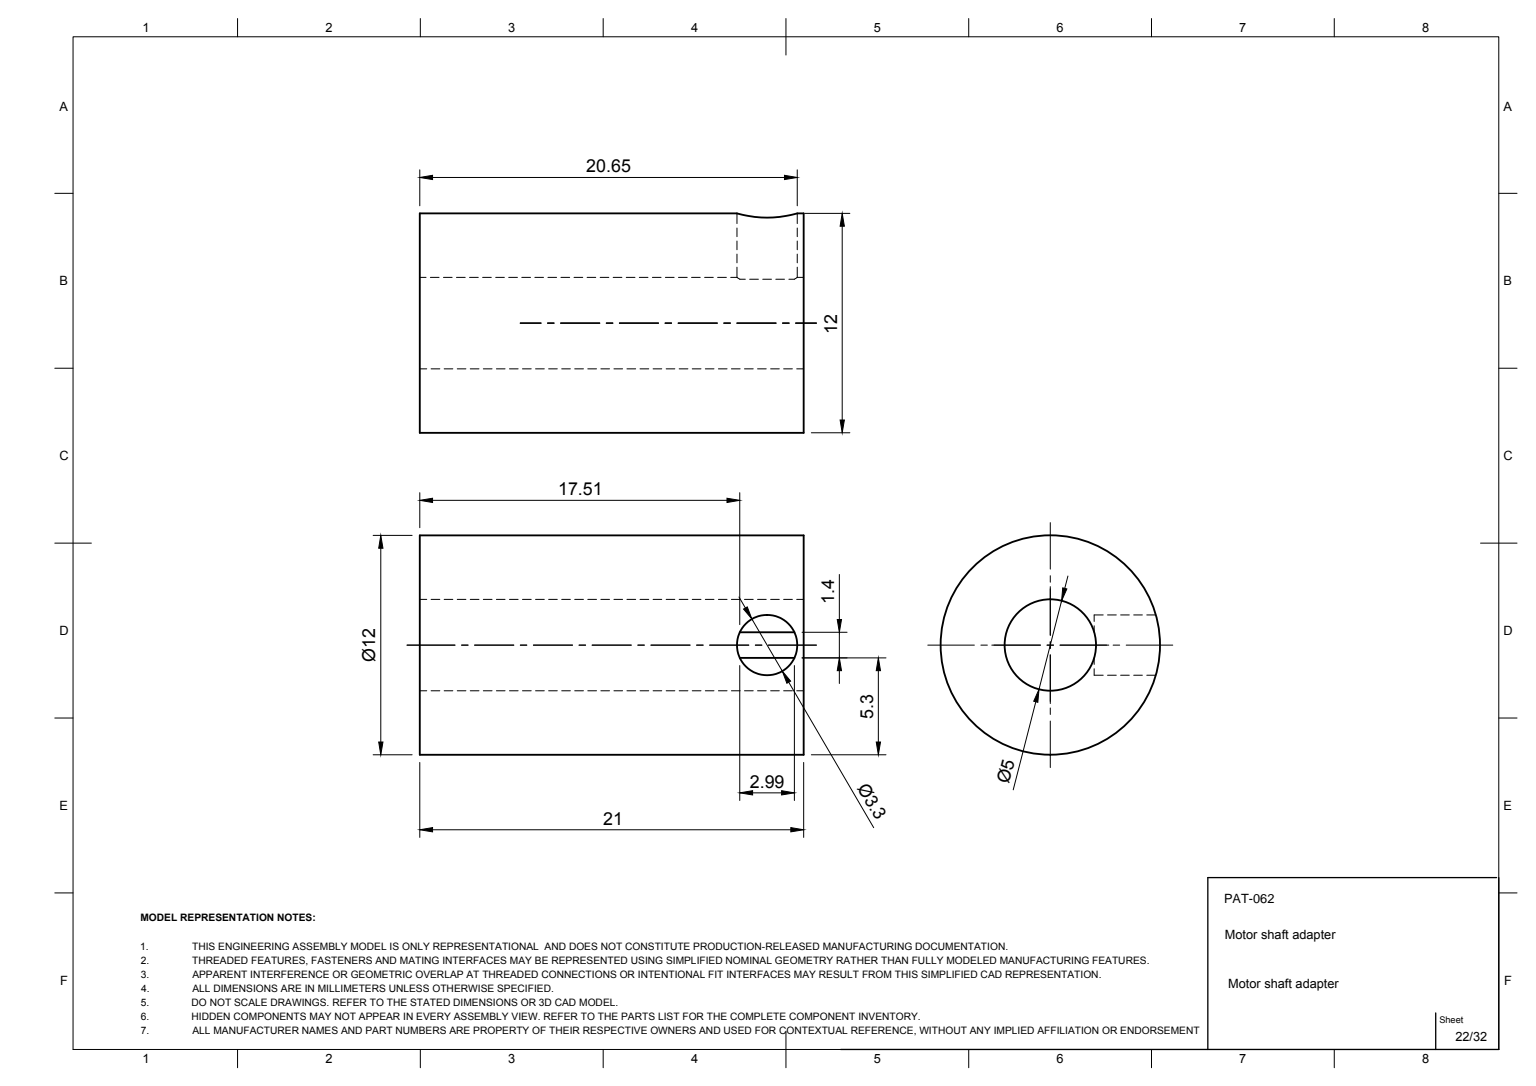
ISO-10303-21;
HEADER;
/* Generated by software containing ST-Developer
 * from STEP Tools, Inc. (www.steptools.com) 
 */

FILE_DESCRIPTION(
/* description */ ('Jaw-coupled motor to shaft test stand'),
/* implementation_level */ '2;1');

FILE_NAME(
/* name */ 'Motor shaft adapter.step',
/* time_stamp */ '2026-10-27T10:46:06-07:00',
/* author */ (''),
/* organization */ (''),
/* preprocessor_version */ 'ST-DEVELOPER v20.2',
/* originating_system */ 'Autodesk Translation Framework v15.17.0.0',
/* authorisation */ '');

FILE_SCHEMA (('AUTOMOTIVE_DESIGN { 1 0 10303 214 3 1 1 }'));
ENDSEC;

DATA;
#10=MECHANICAL_DESIGN_GEOMETRIC_PRESENTATION_REPRESENTATION('',(#361),#19361);
#251=B_SPLINE_CURVE_WITH_KNOTS('',3,(#16870,#16871,#16872,#16873,#16874,
#16875,#16876,#16877,#16878,#16879),.UNSPECIFIED.,.F.,.F.,(4,2,2,2,4),(0.705412572778712,
0.711709336094043,0.776040013313971,0.840370690533898,0.846667453849229),
 .UNSPECIFIED.);
#252=B_SPLINE_CURVE_WITH_KNOTS('',3,(#16885,#16886,#16887,#16888,#16889,
#16890,#16891,#16892,#16893,#16894,#16895,#16896,#16897,#16898,#16899,#16900,
#16901,#16902),.UNSPECIFIED.,.F.,.F.,(4,2,2,2,2,2,2,2,4),(0.,0.0625085224334669,
0.125017044866934,0.187512605393579,0.250008165920225,0.312503726446871,
0.374999286973516,0.437507809406983,0.50001633184045),.UNSPECIFIED.);
#253=B_SPLINE_CURVE_WITH_KNOTS('',3,(#16903,#16904,#16905,#16906,#16907,
#16908,#16909,#16910,#16911,#16912,#16913,#16914,#16915,#16916,#16917,#16918,
#16919,#16920),.UNSPECIFIED.,.F.,.F.,(4,2,2,2,2,2,2,2,4),(0.50001633184045,
0.562524854273917,0.625033376707384,0.687528937234029,0.750024497760675,
0.81252005828732,0.875015618813966,0.937524141247433,1.0000326636809),
 .UNSPECIFIED.);
#254=B_SPLINE_CURVE_WITH_KNOTS('',3,(#16923,#16924,#16925,#16926,#16927,
#16928,#16929,#16930,#16931,#16932),.UNSPECIFIED.,.F.,.F.,(4,2,2,2,4),(0.188052563902732,
0.194349327218063,0.25868000443799,0.323010681657918,0.329307444973249),
 .UNSPECIFIED.);
#296=SHAPE_REPRESENTATION_RELATIONSHIP('SRR','None',#19512,#328);
#328=ADVANCED_BREP_SHAPE_REPRESENTATION('',(#392),#19348);
#361=STYLED_ITEM('',(#19746),#392);
#392=MANIFOLD_SOLID_BREP('Body1',#11007);
#485=FACE_BOUND('',#1942,.T.);
#486=FACE_BOUND('',#1944,.T.);
#487=FACE_BOUND('',#1946,.T.);
#488=FACE_BOUND('',#1948,.T.);
#662=PLANE('',#11767);
#663=PLANE('',#11772);
#664=PLANE('',#11779);
#665=PLANE('',#11780);
#1236=FACE_OUTER_BOUND('',#1938,.T.);
#1237=FACE_OUTER_BOUND('',#1939,.T.);
#1238=FACE_OUTER_BOUND('',#1940,.T.);
#1239=FACE_OUTER_BOUND('',#1941,.T.);
#1240=FACE_OUTER_BOUND('',#1943,.T.);
#1241=FACE_OUTER_BOUND('',#1945,.T.);
#1242=FACE_OUTER_BOUND('',#1947,.T.);
#1938=EDGE_LOOP('',(#8254,#8255));
#1939=EDGE_LOOP('',(#8256,#8257,#8258,#8259,#8260,#8261,#8262,#8263,#8264));
#1940=EDGE_LOOP('',(#8265,#8266,#8267));
#1941=EDGE_LOOP('',(#8268,#8269,#8270,#8271));
#1942=EDGE_LOOP('',(#8272,#8273,#8274,#8275));
#1943=EDGE_LOOP('',(#8276,#8277,#8278,#8279));
#1944=EDGE_LOOP('',(#8280,#8281));
#1945=EDGE_LOOP('',(#8282));
#1946=EDGE_LOOP('',(#8283));
#1947=EDGE_LOOP('',(#8284));
#1948=EDGE_LOOP('',(#8285));
#2677=LINE('',#16866,#3830);
#2678=LINE('',#16883,#3831);
#2679=LINE('',#16934,#3832);
#2680=LINE('',#16939,#3833);
#2681=LINE('',#16945,#3834);
#3830=VECTOR('',#13432,1.);
#3831=VECTOR('',#13439,0.165);
#3832=VECTOR('',#13444,1.);
#3833=VECTOR('',#13449,0.25);
#3834=VECTOR('',#13456,0.6);
#4809=CIRCLE('',#11768,0.165);
#4810=CIRCLE('',#11770,0.165);
#4811=CIRCLE('',#11771,0.165);
#4812=CIRCLE('',#11774,0.25);
#4813=CIRCLE('',#11775,0.25);
#4814=CIRCLE('',#11777,0.6);
#4815=CIRCLE('',#11778,0.6);
#5251=VERTEX_POINT('',#16864);
#5252=VERTEX_POINT('',#16865);
#5253=VERTEX_POINT('',#16869);
#5254=VERTEX_POINT('',#16880);
#5255=VERTEX_POINT('',#16882);
#5256=VERTEX_POINT('',#16884);
#5257=VERTEX_POINT('',#16921);
#5258=VERTEX_POINT('',#16936);
#5259=VERTEX_POINT('',#16938);
#5260=VERTEX_POINT('',#16942);
#5261=VERTEX_POINT('',#16944);
#6338=EDGE_CURVE('',#5251,#5252,#2677,.T.);
#6339=EDGE_CURVE('',#5251,#5252,#4809,.T.);
#6340=EDGE_CURVE('',#5253,#5251,#251,.T.);
#6341=EDGE_CURVE('',#5254,#5253,#4810,.T.);
#6342=EDGE_CURVE('',#5254,#5255,#2678,.T.);
#6343=EDGE_CURVE('',#5256,#5255,#252,.T.);
#6344=EDGE_CURVE('',#5255,#5256,#253,.T.);
#6345=EDGE_CURVE('',#5257,#5254,#4811,.T.);
#6346=EDGE_CURVE('',#5252,#5257,#254,.T.);
#6347=EDGE_CURVE('',#5257,#5253,#2679,.T.);
#6348=EDGE_CURVE('',#5258,#5258,#4812,.T.);
#6349=EDGE_CURVE('',#5258,#5259,#2680,.T.);
#6350=EDGE_CURVE('',#5259,#5259,#4813,.T.);
#6351=EDGE_CURVE('',#5260,#5260,#4814,.T.);
#6352=EDGE_CURVE('',#5260,#5261,#2681,.T.);
#6353=EDGE_CURVE('',#5261,#5261,#4815,.T.);
#8254=ORIENTED_EDGE('',*,*,#6338,.F.);
#8255=ORIENTED_EDGE('',*,*,#6339,.T.);
#8256=ORIENTED_EDGE('',*,*,#6340,.F.);
#8257=ORIENTED_EDGE('',*,*,#6341,.F.);
#8258=ORIENTED_EDGE('',*,*,#6342,.T.);
#8259=ORIENTED_EDGE('',*,*,#6343,.F.);
#8260=ORIENTED_EDGE('',*,*,#6344,.F.);
#8261=ORIENTED_EDGE('',*,*,#6342,.F.);
#8262=ORIENTED_EDGE('',*,*,#6345,.F.);
#8263=ORIENTED_EDGE('',*,*,#6346,.F.);
#8264=ORIENTED_EDGE('',*,*,#6339,.F.);
#8265=ORIENTED_EDGE('',*,*,#6347,.F.);
#8266=ORIENTED_EDGE('',*,*,#6345,.T.);
#8267=ORIENTED_EDGE('',*,*,#6341,.T.);
#8268=ORIENTED_EDGE('',*,*,#6348,.F.);
#8269=ORIENTED_EDGE('',*,*,#6349,.T.);
#8270=ORIENTED_EDGE('',*,*,#6350,.T.);
#8271=ORIENTED_EDGE('',*,*,#6349,.F.);
#8272=ORIENTED_EDGE('',*,*,#6346,.T.);
#8273=ORIENTED_EDGE('',*,*,#6347,.T.);
#8274=ORIENTED_EDGE('',*,*,#6340,.T.);
#8275=ORIENTED_EDGE('',*,*,#6338,.T.);
#8276=ORIENTED_EDGE('',*,*,#6351,.F.);
#8277=ORIENTED_EDGE('',*,*,#6352,.T.);
#8278=ORIENTED_EDGE('',*,*,#6353,.T.);
#8279=ORIENTED_EDGE('',*,*,#6352,.F.);
#8280=ORIENTED_EDGE('',*,*,#6343,.T.);
#8281=ORIENTED_EDGE('',*,*,#6344,.T.);
#8282=ORIENTED_EDGE('',*,*,#6351,.T.);
#8283=ORIENTED_EDGE('',*,*,#6348,.T.);
#8284=ORIENTED_EDGE('',*,*,#6353,.F.);
#8285=ORIENTED_EDGE('',*,*,#6350,.F.);
#10330=CYLINDRICAL_SURFACE('',#11769,0.165);
#10331=CYLINDRICAL_SURFACE('',#11773,0.25);
#10332=CYLINDRICAL_SURFACE('',#11776,0.6);
#10578=ADVANCED_FACE('',(#1236),#662,.T.);
#10579=ADVANCED_FACE('',(#1237),#10330,.F.);
#10580=ADVANCED_FACE('',(#1238),#663,.T.);
#10581=ADVANCED_FACE('',(#1239,#485),#10331,.F.);
#10582=ADVANCED_FACE('',(#1240,#486),#10332,.T.);
#10583=ADVANCED_FACE('',(#1241,#487),#664,.T.);
#10584=ADVANCED_FACE('',(#1242,#488),#665,.F.);
#11007=CLOSED_SHELL('',(#10578,#10579,#10580,#10581,#10582,#10583,#10584));
#11766=AXIS2_PLACEMENT_3D('',#16862,#13428,#13429);
#11767=AXIS2_PLACEMENT_3D('',#16863,#13430,#13431);
#11768=AXIS2_PLACEMENT_3D('',#16867,#13433,#13434);
#11769=AXIS2_PLACEMENT_3D('',#16868,#13435,#13436);
#11770=AXIS2_PLACEMENT_3D('',#16881,#13437,#13438);
#11771=AXIS2_PLACEMENT_3D('',#16922,#13440,#13441);
#11772=AXIS2_PLACEMENT_3D('',#16933,#13442,#13443);
#11773=AXIS2_PLACEMENT_3D('',#16935,#13445,#13446);
#11774=AXIS2_PLACEMENT_3D('',#16937,#13447,#13448);
#11775=AXIS2_PLACEMENT_3D('',#16940,#13450,#13451);
#11776=AXIS2_PLACEMENT_3D('',#16941,#13452,#13453);
#11777=AXIS2_PLACEMENT_3D('',#16943,#13454,#13455);
#11778=AXIS2_PLACEMENT_3D('',#16946,#13457,#13458);
#11779=AXIS2_PLACEMENT_3D('',#16947,#13459,#13460);
#11780=AXIS2_PLACEMENT_3D('',#16948,#13461,#13462);
#13428=DIRECTION('axis',(0.,0.,1.));
#13429=DIRECTION('refdir',(1.,0.,0.));
#13430=DIRECTION('center_axis',(0.,0.,1.));
#13431=DIRECTION('ref_axis',(1.,0.,0.));
#13432=DIRECTION('',(0.,1.,0.));
#13433=DIRECTION('center_axis',(0.,0.,1.));
#13434=DIRECTION('ref_axis',(1.,0.,0.));
#13435=DIRECTION('center_axis',(0.,0.,1.));
#13436=DIRECTION('ref_axis',(1.,0.,0.));
#13437=DIRECTION('center_axis',(0.,0.,1.));
#13438=DIRECTION('ref_axis',(1.,0.,0.));
#13439=DIRECTION('',(0.,0.,1.));
#13440=DIRECTION('center_axis',(0.,0.,1.));
#13441=DIRECTION('ref_axis',(1.,0.,0.));
#13442=DIRECTION('center_axis',(0.,0.,1.));
#13443=DIRECTION('ref_axis',(1.,0.,0.));
#13444=DIRECTION('',(0.,-1.,0.));
#13445=DIRECTION('center_axis',(0.,1.,0.));
#13446=DIRECTION('ref_axis',(1.,0.,0.));
#13447=DIRECTION('center_axis',(0.,-1.,0.));
#13448=DIRECTION('ref_axis',(1.,0.,0.));
#13449=DIRECTION('',(0.,-1.,0.));
#13450=DIRECTION('center_axis',(0.,-1.,0.));
#13451=DIRECTION('ref_axis',(1.,0.,0.));
#13452=DIRECTION('center_axis',(0.,1.,0.));
#13453=DIRECTION('ref_axis',(1.,0.,0.));
#13454=DIRECTION('center_axis',(0.,1.,0.));
#13455=DIRECTION('ref_axis',(1.,0.,0.));
#13456=DIRECTION('',(0.,-1.,0.));
#13457=DIRECTION('center_axis',(0.,1.,0.));
#13458=DIRECTION('ref_axis',(1.,0.,0.));
#13459=DIRECTION('center_axis',(0.,1.,0.));
#13460=DIRECTION('ref_axis',(1.,0.,0.));
#13461=DIRECTION('center_axis',(0.,1.,0.));
#13462=DIRECTION('ref_axis',(1.,0.,0.));
#16862=CARTESIAN_POINT('',(0.,0.,0.));
#16863=CARTESIAN_POINT('Origin',(0.,-5.8,4.46));
#16864=CARTESIAN_POINT('',(0.0700000000000023,-5.94941552797484,4.46));
#16865=CARTESIAN_POINT('',(0.0700000000000023,-5.65058447202516,4.46));
#16866=CARTESIAN_POINT('',(0.0700000000000023,-6.,4.46));
#16867=CARTESIAN_POINT('Origin',(0.,-5.8,4.46));
#16868=CARTESIAN_POINT('Origin',(0.,-5.8,4.46));
#16869=CARTESIAN_POINT('',(-0.0700000000000023,-5.94941552797484,4.46));
#16870=CARTESIAN_POINT('Ctrl Pts',(-0.0700000000000023,-5.94941552797484,
4.46));
#16871=CARTESIAN_POINT('Ctrl Pts',(-0.06805939906088,-5.95032468425585,
4.46056600860724));
#16872=CARTESIAN_POINT('Ctrl Pts',(-0.0660971141771659,-5.95119787419286,
4.46111278532807));
#16873=CARTESIAN_POINT('Ctrl Pts',(-0.0438689676213799,-5.9605718962209,
4.4670107091875));
#16874=CARTESIAN_POINT('Ctrl Pts',(-0.0214435590733092,-5.965,4.47));
#16875=CARTESIAN_POINT('Ctrl Pts',(0.0214435590733092,-5.965,4.47));
#16876=CARTESIAN_POINT('Ctrl Pts',(0.0438689676213799,-5.9605718962209,
4.4670107091875));
#16877=CARTESIAN_POINT('Ctrl Pts',(0.0660971141771659,-5.95119787419286,
4.46111278532807));
#16878=CARTESIAN_POINT('Ctrl Pts',(0.06805939906088,-5.95032468425585,4.46056600860724));
#16879=CARTESIAN_POINT('Ctrl Pts',(0.0700000000000023,-5.94941552797484,
4.46));
#16880=CARTESIAN_POINT('',(-0.165,-5.8,4.46));
#16881=CARTESIAN_POINT('Origin',(0.,-5.8,4.46));
#16882=CARTESIAN_POINT('',(-0.165,-5.8,4.79686653569088));
#16883=CARTESIAN_POINT('',(-0.165,-5.8,4.46));
#16884=CARTESIAN_POINT('',(0.165,-5.8,4.79686653569088));
#16885=CARTESIAN_POINT('Ctrl Pts',(0.165,-5.8,4.79686653569088));
#16886=CARTESIAN_POINT('Ctrl Pts',(0.165,-5.82083617414449,4.79686653569088));
#16887=CARTESIAN_POINT('Ctrl Pts',(0.160813813148411,-5.84298285479422,
4.79811329537163));
#16888=CARTESIAN_POINT('Ctrl Pts',(0.143942819671378,-5.88360069371169,
4.80254315455331));
#16889=CARTESIAN_POINT('Ctrl Pts',(0.13126336772609,-5.90208187006547,4.80565449242259));
#16890=CARTESIAN_POINT('Ctrl Pts',(0.102084895635736,-5.93126034215582,
4.81143878680194));
#16891=CARTESIAN_POINT('Ctrl Pts',(0.0836024737060978,-5.9439421456793,
4.81449794909247));
#16892=CARTESIAN_POINT('Ctrl Pts',(0.0429801659601906,-5.96081486463402,
4.81880705606552));
#16893=CARTESIAN_POINT('Ctrl Pts',(0.0208318535088818,-5.965,4.82));
#16894=CARTESIAN_POINT('Ctrl Pts',(-0.0208318535088819,-5.965,4.82));
#16895=CARTESIAN_POINT('Ctrl Pts',(-0.0429801659601906,-5.96081486463402,
4.81880705606552));
#16896=CARTESIAN_POINT('Ctrl Pts',(-0.0836024737060979,-5.9439421456793,
4.81449794909247));
#16897=CARTESIAN_POINT('Ctrl Pts',(-0.102084895635736,-5.93126034215582,
4.81143878680194));
#16898=CARTESIAN_POINT('Ctrl Pts',(-0.13126336772609,-5.90208187006547,
4.80565449242259));
#16899=CARTESIAN_POINT('Ctrl Pts',(-0.143942819671378,-5.88360069371169,
4.80254315455331));
#16900=CARTESIAN_POINT('Ctrl Pts',(-0.160813813148411,-5.84298285479422,
4.79811329537163));
#16901=CARTESIAN_POINT('Ctrl Pts',(-0.165,-5.82083617414449,4.79686653569088));
#16902=CARTESIAN_POINT('Ctrl Pts',(-0.165,-5.8,4.79686653569088));
#16903=CARTESIAN_POINT('Ctrl Pts',(-0.165,-5.8,4.79686653569088));
#16904=CARTESIAN_POINT('Ctrl Pts',(-0.165,-5.77916382585551,4.79686653569088));
#16905=CARTESIAN_POINT('Ctrl Pts',(-0.160813813148411,-5.75701714520578,
4.79811329537163));
#16906=CARTESIAN_POINT('Ctrl Pts',(-0.143942819671378,-5.71639930628831,
4.80254315455331));
#16907=CARTESIAN_POINT('Ctrl Pts',(-0.13126336772609,-5.69791812993453,
4.80565449242259));
#16908=CARTESIAN_POINT('Ctrl Pts',(-0.102084895635736,-5.66873965784418,
4.81143878680194));
#16909=CARTESIAN_POINT('Ctrl Pts',(-0.0836024737060979,-5.6560578543207,
4.81449794909247));
#16910=CARTESIAN_POINT('Ctrl Pts',(-0.0429801659601906,-5.63918513536598,
4.81880705606552));
#16911=CARTESIAN_POINT('Ctrl Pts',(-0.0208318535088819,-5.635,4.82));
#16912=CARTESIAN_POINT('Ctrl Pts',(0.0208318535088818,-5.635,4.82));
#16913=CARTESIAN_POINT('Ctrl Pts',(0.0429801659601906,-5.63918513536598,
4.81880705606552));
#16914=CARTESIAN_POINT('Ctrl Pts',(0.0836024737060978,-5.6560578543207,
4.81449794909247));
#16915=CARTESIAN_POINT('Ctrl Pts',(0.102084895635736,-5.66873965784418,
4.81143878680194));
#16916=CARTESIAN_POINT('Ctrl Pts',(0.13126336772609,-5.69791812993453,4.80565449242259));
#16917=CARTESIAN_POINT('Ctrl Pts',(0.143942819671378,-5.71639930628831,
4.80254315455331));
#16918=CARTESIAN_POINT('Ctrl Pts',(0.160813813148411,-5.75701714520578,
4.79811329537163));
#16919=CARTESIAN_POINT('Ctrl Pts',(0.165,-5.77916382585551,4.79686653569088));
#16920=CARTESIAN_POINT('Ctrl Pts',(0.165,-5.8,4.79686653569088));
#16921=CARTESIAN_POINT('',(-0.0700000000000023,-5.65058447202516,4.46));
#16922=CARTESIAN_POINT('Origin',(0.,-5.8,4.46));
#16923=CARTESIAN_POINT('Ctrl Pts',(0.0700000000000023,-5.65058447202516,
4.46));
#16924=CARTESIAN_POINT('Ctrl Pts',(0.0680593990608798,-5.64967531574415,
4.46056600860724));
#16925=CARTESIAN_POINT('Ctrl Pts',(0.0660971141771658,-5.64880212580714,
4.46111278532807));
#16926=CARTESIAN_POINT('Ctrl Pts',(0.0438689676213798,-5.6394281037791,
4.4670107091875));
#16927=CARTESIAN_POINT('Ctrl Pts',(0.0214435590733091,-5.635,4.47));
#16928=CARTESIAN_POINT('Ctrl Pts',(-0.0214435590733092,-5.635,4.47));
#16929=CARTESIAN_POINT('Ctrl Pts',(-0.0438689676213799,-5.6394281037791,
4.4670107091875));
#16930=CARTESIAN_POINT('Ctrl Pts',(-0.0660971141771659,-5.64880212580714,
4.46111278532807));
#16931=CARTESIAN_POINT('Ctrl Pts',(-0.0680593990608798,-5.64967531574415,
4.46056600860724));
#16932=CARTESIAN_POINT('Ctrl Pts',(-0.0700000000000023,-5.65058447202516,
4.46));
#16933=CARTESIAN_POINT('Origin',(0.,-5.8,4.46));
#16934=CARTESIAN_POINT('',(-0.0700000000000023,-6.,4.46));
#16935=CARTESIAN_POINT('Origin',(0.,-6.,4.22));
#16936=CARTESIAN_POINT('',(-0.25,-3.9,4.22));
#16937=CARTESIAN_POINT('Origin',(0.,-3.9,4.22));
#16938=CARTESIAN_POINT('',(-0.25,-6.,4.22));
#16939=CARTESIAN_POINT('',(-0.25,-6.,4.22));
#16940=CARTESIAN_POINT('Origin',(0.,-6.,4.22));
#16941=CARTESIAN_POINT('Origin',(0.,-6.,4.22));
#16942=CARTESIAN_POINT('',(-0.6,-3.9,4.22));
#16943=CARTESIAN_POINT('Origin',(0.,-3.9,4.22));
#16944=CARTESIAN_POINT('',(-0.6,-6.,4.22));
#16945=CARTESIAN_POINT('',(-0.6,-6.,4.22));
#16946=CARTESIAN_POINT('Origin',(0.,-6.,4.22));
#16947=CARTESIAN_POINT('Origin',(0.,-3.9,4.22));
#16948=CARTESIAN_POINT('Origin',(0.,-6.,4.22));
#19310=UNCERTAINTY_MEASURE_WITH_UNIT(LENGTH_MEASURE(0.001),#19362,
'DISTANCE_ACCURACY_VALUE',
'Maximum model space distance between geometric entities at asserted c
onnectivities');
#19323=UNCERTAINTY_MEASURE_WITH_UNIT(LENGTH_MEASURE(0.001),#19362,
'DISTANCE_ACCURACY_VALUE',
'Maximum model space distance between geometric entities at asserted c
onnectivities');
#19348=(
GEOMETRIC_REPRESENTATION_CONTEXT(3)
GLOBAL_UNCERTAINTY_ASSIGNED_CONTEXT((#19310))
GLOBAL_UNIT_ASSIGNED_CONTEXT((#19362,#19364,#19365))
REPRESENTATION_CONTEXT('','3D')
);
#19361=(
GEOMETRIC_REPRESENTATION_CONTEXT(3)
GLOBAL_UNCERTAINTY_ASSIGNED_CONTEXT((#19323))
GLOBAL_UNIT_ASSIGNED_CONTEXT((#19362,#19364,#19365))
REPRESENTATION_CONTEXT('','3D')
);
#19362=(
LENGTH_UNIT()
NAMED_UNIT(*)
SI_UNIT(.CENTI.,.METRE.)
);
#19364=(
NAMED_UNIT(*)
PLANE_ANGLE_UNIT()
SI_UNIT($,.RADIAN.)
);
#19365=(
NAMED_UNIT(*)
SI_UNIT($,.STERADIAN.)
SOLID_ANGLE_UNIT()
);
#19390=SHAPE_DEFINITION_REPRESENTATION(#19454,#19512);
#19454=PRODUCT_DEFINITION_SHAPE('',$,#19550);
#19512=SHAPE_REPRESENTATION('',(#11766),#19348);
#19525=PRODUCT_DEFINITION_CONTEXT('part definition',#19638,'design');
#19550=PRODUCT_DEFINITION('Motor shaft adapter','Motor shaft adapter',#19587,
#19525);
#19587=PRODUCT_DEFINITION_FORMATION('',$,#19664);
#19638=APPLICATION_CONTEXT(
'Core Data for Automotive Mechanical Design Process');
#19639=PRODUCT_CONTEXT('part definition',#19638,'mechanical');
#19664=PRODUCT('Motor shaft adapter','Motor shaft adapter',
'Motor shaft adapter',(#19639));
#19740=COLOUR_RGB('Grey',0.48,0.52,0.57);
#19741=FILL_AREA_STYLE_COLOUR('',#19740);
#19742=FILL_AREA_STYLE('',(#19741));
#19743=SURFACE_STYLE_FILL_AREA(#19742);
#19744=SURFACE_SIDE_STYLE('',(#19743));
#19745=SURFACE_STYLE_USAGE(.BOTH.,#19744);
#19746=PRESENTATION_STYLE_ASSIGNMENT((#19745));
ENDSEC;
END-ISO-10303-21;
